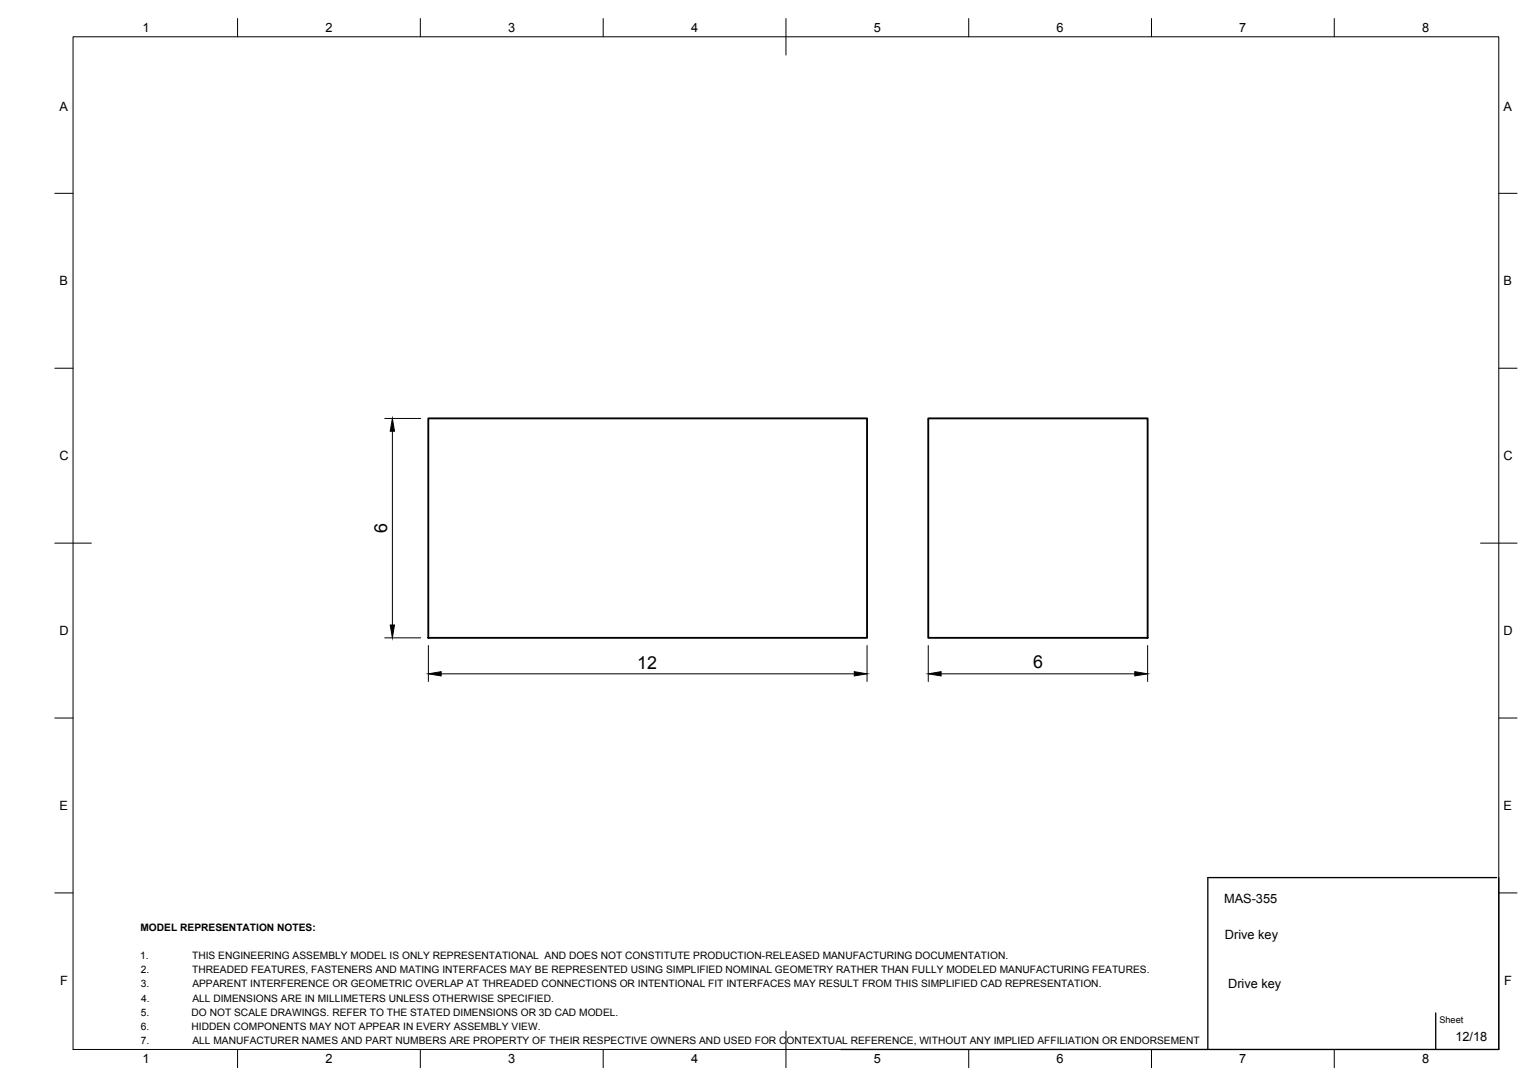
ISO-10303-21;
HEADER;
/* Generated by software containing ST-Developer
 * from STEP Tools, Inc. (www.steptools.com) 
 */

FILE_DESCRIPTION(
/* description */ ('Independent two-stage fixed-ring planetary gearbox,24/24/72 teeth,mod
ule2,20deg involutes,three planets per stage,4:1 x4:1=16:1. Native cut
-space/fillet/pattern tooth profiles derived from reusable gear blanks
; shared sun/planet/ring/carrier parts across both stages. Captured br
onze-journal input/carriers, headed retained planet pins, keyed inters
tage drive and modular keyed output interface. Native ideal gear links
; no torque, precision grade, production backlash/fits, lubrication, s
peed or life rating.'),
/* implementation_level */ '2;1');

FILE_NAME(
/* name */ 'Drive key.step',
/* time_stamp */ '2026-11-08T19:10:00-08:00',
/* author */ (''),
/* organization */ (''),
/* preprocessor_version */ 'ST-DEVELOPER v20.2',
/* originating_system */ 'Autodesk Translation Framework v15.17.0.0',
/* authorisation */ '');

FILE_SCHEMA (('AUTOMOTIVE_DESIGN { 1 0 10303 214 3 1 1 }'));
ENDSEC;

DATA;
#10=MECHANICAL_DESIGN_GEOMETRIC_PRESENTATION_REPRESENTATION('',(#1172),#259224);
#1132=SHAPE_REPRESENTATION_RELATIONSHIP('SRR','None',#259379,#1152);
#1152=ADVANCED_BREP_SHAPE_REPRESENTATION('',(#1192),#259213);
#1172=STYLED_ITEM('',(#259487),#1192);
#1192=MANIFOLD_SOLID_BREP('Body1',#25159);
#1655=PLANE('',#27077);
#1656=PLANE('',#27078);
#1657=PLANE('',#27079);
#1658=PLANE('',#27080);
#1659=PLANE('',#27081);
#1660=PLANE('',#27082);
#2937=FACE_OUTER_BOUND('',#4385,.T.);
#2938=FACE_OUTER_BOUND('',#4386,.T.);
#2939=FACE_OUTER_BOUND('',#4387,.T.);
#2940=FACE_OUTER_BOUND('',#4388,.T.);
#2941=FACE_OUTER_BOUND('',#4389,.T.);
#2942=FACE_OUTER_BOUND('',#4390,.T.);
#4385=EDGE_LOOP('',(#22598,#22599,#22600,#22601));
#4386=EDGE_LOOP('',(#22602,#22603,#22604,#22605));
#4387=EDGE_LOOP('',(#22606,#22607,#22608,#22609));
#4388=EDGE_LOOP('',(#22610,#22611,#22612,#22613));
#4389=EDGE_LOOP('',(#22614,#22615,#22616,#22617));
#4390=EDGE_LOOP('',(#22618,#22619,#22620,#22621));
#7744=LINE('',#255905,#8929);
#7745=LINE('',#255907,#8930);
#7746=LINE('',#255909,#8931);
#7747=LINE('',#255910,#8932);
#7748=LINE('',#255913,#8933);
#7749=LINE('',#255915,#8934);
#7750=LINE('',#255916,#8935);
#7751=LINE('',#255919,#8936);
#7752=LINE('',#255921,#8937);
#7753=LINE('',#255922,#8938);
#7754=LINE('',#255924,#8939);
#7755=LINE('',#255925,#8940);
#8929=VECTOR('',#31785,10.);
#8930=VECTOR('',#31786,10.);
#8931=VECTOR('',#31787,10.);
#8932=VECTOR('',#31788,10.);
#8933=VECTOR('',#31791,10.);
#8934=VECTOR('',#31792,10.);
#8935=VECTOR('',#31793,10.);
#8936=VECTOR('',#31796,10.);
#8937=VECTOR('',#31797,10.);
#8938=VECTOR('',#31798,10.);
#8939=VECTOR('',#31801,10.);
#8940=VECTOR('',#31802,10.);
#11437=VERTEX_POINT('',#255903);
#11438=VERTEX_POINT('',#255904);
#11439=VERTEX_POINT('',#255906);
#11440=VERTEX_POINT('',#255908);
#11441=VERTEX_POINT('',#255912);
#11442=VERTEX_POINT('',#255914);
#11443=VERTEX_POINT('',#255918);
#11444=VERTEX_POINT('',#255920);
#15184=EDGE_CURVE('',#11437,#11438,#7744,.T.);
#15185=EDGE_CURVE('',#11438,#11439,#7745,.T.);
#15186=EDGE_CURVE('',#11440,#11439,#7746,.T.);
#15187=EDGE_CURVE('',#11437,#11440,#7747,.T.);
#15188=EDGE_CURVE('',#11441,#11437,#7748,.T.);
#15189=EDGE_CURVE('',#11442,#11440,#7749,.T.);
#15190=EDGE_CURVE('',#11441,#11442,#7750,.T.);
#15191=EDGE_CURVE('',#11443,#11441,#7751,.T.);
#15192=EDGE_CURVE('',#11444,#11442,#7752,.T.);
#15193=EDGE_CURVE('',#11443,#11444,#7753,.T.);
#15194=EDGE_CURVE('',#11438,#11443,#7754,.T.);
#15195=EDGE_CURVE('',#11439,#11444,#7755,.T.);
#22598=ORIENTED_EDGE('',*,*,#15184,.T.);
#22599=ORIENTED_EDGE('',*,*,#15185,.T.);
#22600=ORIENTED_EDGE('',*,*,#15186,.F.);
#22601=ORIENTED_EDGE('',*,*,#15187,.F.);
#22602=ORIENTED_EDGE('',*,*,#15188,.T.);
#22603=ORIENTED_EDGE('',*,*,#15187,.T.);
#22604=ORIENTED_EDGE('',*,*,#15189,.F.);
#22605=ORIENTED_EDGE('',*,*,#15190,.F.);
#22606=ORIENTED_EDGE('',*,*,#15191,.T.);
#22607=ORIENTED_EDGE('',*,*,#15190,.T.);
#22608=ORIENTED_EDGE('',*,*,#15192,.F.);
#22609=ORIENTED_EDGE('',*,*,#15193,.F.);
#22610=ORIENTED_EDGE('',*,*,#15194,.T.);
#22611=ORIENTED_EDGE('',*,*,#15193,.T.);
#22612=ORIENTED_EDGE('',*,*,#15195,.F.);
#22613=ORIENTED_EDGE('',*,*,#15185,.F.);
#22614=ORIENTED_EDGE('',*,*,#15195,.T.);
#22615=ORIENTED_EDGE('',*,*,#15192,.T.);
#22616=ORIENTED_EDGE('',*,*,#15189,.T.);
#22617=ORIENTED_EDGE('',*,*,#15186,.T.);
#22618=ORIENTED_EDGE('',*,*,#15194,.F.);
#22619=ORIENTED_EDGE('',*,*,#15184,.F.);
#22620=ORIENTED_EDGE('',*,*,#15188,.F.);
#22621=ORIENTED_EDGE('',*,*,#15191,.F.);
#25043=ADVANCED_FACE('',(#2937),#1655,.T.);
#25044=ADVANCED_FACE('',(#2938),#1656,.T.);
#25045=ADVANCED_FACE('',(#2939),#1657,.T.);
#25046=ADVANCED_FACE('',(#2940),#1658,.T.);
#25047=ADVANCED_FACE('',(#2941),#1659,.T.);
#25048=ADVANCED_FACE('',(#2942),#1660,.F.);
#25159=CLOSED_SHELL('',(#25043,#25044,#25045,#25046,#25047,#25048));
#27076=AXIS2_PLACEMENT_3D('',#255901,#31781,#31782);
#27077=AXIS2_PLACEMENT_3D('',#255902,#31783,#31784);
#27078=AXIS2_PLACEMENT_3D('',#255911,#31789,#31790);
#27079=AXIS2_PLACEMENT_3D('',#255917,#31794,#31795);
#27080=AXIS2_PLACEMENT_3D('',#255923,#31799,#31800);
#27081=AXIS2_PLACEMENT_3D('',#255926,#31803,#31804);
#27082=AXIS2_PLACEMENT_3D('',#255927,#31805,#31806);
#31781=DIRECTION('axis',(0.,0.,1.));
#31782=DIRECTION('refdir',(1.,0.,0.));
#31783=DIRECTION('center_axis',(0.,1.,0.));
#31784=DIRECTION('ref_axis',(-1.,0.,0.));
#31785=DIRECTION('',(-1.,0.,0.));
#31786=DIRECTION('',(0.,0.,1.));
#31787=DIRECTION('',(-1.,0.,0.));
#31788=DIRECTION('',(0.,0.,1.));
#31789=DIRECTION('center_axis',(1.,0.,0.));
#31790=DIRECTION('ref_axis',(0.,1.,0.));
#31791=DIRECTION('',(0.,1.,0.));
#31792=DIRECTION('',(0.,1.,0.));
#31793=DIRECTION('',(0.,0.,1.));
#31794=DIRECTION('center_axis',(0.,-1.,0.));
#31795=DIRECTION('ref_axis',(1.,0.,0.));
#31796=DIRECTION('',(1.,0.,0.));
#31797=DIRECTION('',(1.,0.,0.));
#31798=DIRECTION('',(0.,0.,1.));
#31799=DIRECTION('center_axis',(-1.,0.,0.));
#31800=DIRECTION('ref_axis',(0.,-1.,0.));
#31801=DIRECTION('',(0.,-1.,0.));
#31802=DIRECTION('',(0.,-1.,0.));
#31803=DIRECTION('center_axis',(0.,0.,1.));
#31804=DIRECTION('ref_axis',(1.,0.,0.));
#31805=DIRECTION('center_axis',(0.,0.,1.));
#31806=DIRECTION('ref_axis',(1.,0.,0.));
#255901=CARTESIAN_POINT('',(0.,0.,0.));
#255902=CARTESIAN_POINT('Origin',(11.,3.,0.));
#255903=CARTESIAN_POINT('',(11.,3.,0.));
#255904=CARTESIAN_POINT('',(5.,3.,0.));
#255905=CARTESIAN_POINT('',(11.,3.,0.));
#255906=CARTESIAN_POINT('',(5.,3.,12.));
#255907=CARTESIAN_POINT('',(5.,3.,0.));
#255908=CARTESIAN_POINT('',(11.,3.,12.));
#255909=CARTESIAN_POINT('',(11.,3.,12.));
#255910=CARTESIAN_POINT('',(11.,3.,0.));
#255911=CARTESIAN_POINT('Origin',(11.,-3.,0.));
#255912=CARTESIAN_POINT('',(11.,-3.,0.));
#255913=CARTESIAN_POINT('',(11.,-3.,0.));
#255914=CARTESIAN_POINT('',(11.,-3.,12.));
#255915=CARTESIAN_POINT('',(11.,-3.,12.));
#255916=CARTESIAN_POINT('',(11.,-3.,0.));
#255917=CARTESIAN_POINT('Origin',(5.,-3.,0.));
#255918=CARTESIAN_POINT('',(5.,-3.,0.));
#255919=CARTESIAN_POINT('',(5.,-3.,0.));
#255920=CARTESIAN_POINT('',(5.,-3.,12.));
#255921=CARTESIAN_POINT('',(5.,-3.,12.));
#255922=CARTESIAN_POINT('',(5.,-3.,0.));
#255923=CARTESIAN_POINT('Origin',(5.,3.,0.));
#255924=CARTESIAN_POINT('',(5.,3.,0.));
#255925=CARTESIAN_POINT('',(5.,3.,12.));
#255926=CARTESIAN_POINT('Origin',(8.,0.,12.));
#255927=CARTESIAN_POINT('Origin',(8.,0.,0.));
#259191=UNCERTAINTY_MEASURE_WITH_UNIT(LENGTH_MEASURE(0.01),#259225,
'DISTANCE_ACCURACY_VALUE',
'Maximum model space distance between geometric entities at asserted c
onnectivities');
#259202=UNCERTAINTY_MEASURE_WITH_UNIT(LENGTH_MEASURE(0.01),#259225,
'DISTANCE_ACCURACY_VALUE',
'Maximum model space distance between geometric entities at asserted c
onnectivities');
#259213=(
GEOMETRIC_REPRESENTATION_CONTEXT(3)
GLOBAL_UNCERTAINTY_ASSIGNED_CONTEXT((#259191))
GLOBAL_UNIT_ASSIGNED_CONTEXT((#259225,#259227,#259228))
REPRESENTATION_CONTEXT('','3D')
);
#259224=(
GEOMETRIC_REPRESENTATION_CONTEXT(3)
GLOBAL_UNCERTAINTY_ASSIGNED_CONTEXT((#259202))
GLOBAL_UNIT_ASSIGNED_CONTEXT((#259225,#259227,#259228))
REPRESENTATION_CONTEXT('','3D')
);
#259225=(
LENGTH_UNIT()
NAMED_UNIT(*)
SI_UNIT(.MILLI.,.METRE.)
);
#259227=(
NAMED_UNIT(*)
PLANE_ANGLE_UNIT()
SI_UNIT($,.RADIAN.)
);
#259228=(
NAMED_UNIT(*)
SI_UNIT($,.STERADIAN.)
SOLID_ANGLE_UNIT()
);
#259239=SHAPE_DEFINITION_REPRESENTATION(#259260,#259379);
#259260=PRODUCT_DEFINITION_SHAPE('',$,#259401);
#259379=SHAPE_REPRESENTATION('',(#27076),#259213);
#259390=PRODUCT_DEFINITION_CONTEXT('part definition',#259455,'design');
#259401=PRODUCT_DEFINITION('Drive key','Drive key',#259422,#259390);
#259422=PRODUCT_DEFINITION_FORMATION('',$,#259467);
#259455=APPLICATION_CONTEXT(
'Core Data for Automotive Mechanical Design Process');
#259456=PRODUCT_CONTEXT('part definition',#259455,'mechanical');
#259467=PRODUCT('Drive key','Drive key',$,(#259456));
#259487=PRESENTATION_STYLE_ASSIGNMENT((#259502));
#259502=SURFACE_STYLE_USAGE(.BOTH.,#259517);
#259517=SURFACE_SIDE_STYLE('',(#259532));
#259532=SURFACE_STYLE_FILL_AREA(#259547);
#259547=FILL_AREA_STYLE('Key gray',(#259562));
#259562=FILL_AREA_STYLE_COLOUR('Key gray',#259577);
#259577=COLOUR_RGB('Key gray',0.576470588235294,0.615686274509804,0.666666666666667);
ENDSEC;
END-ISO-10303-21;
